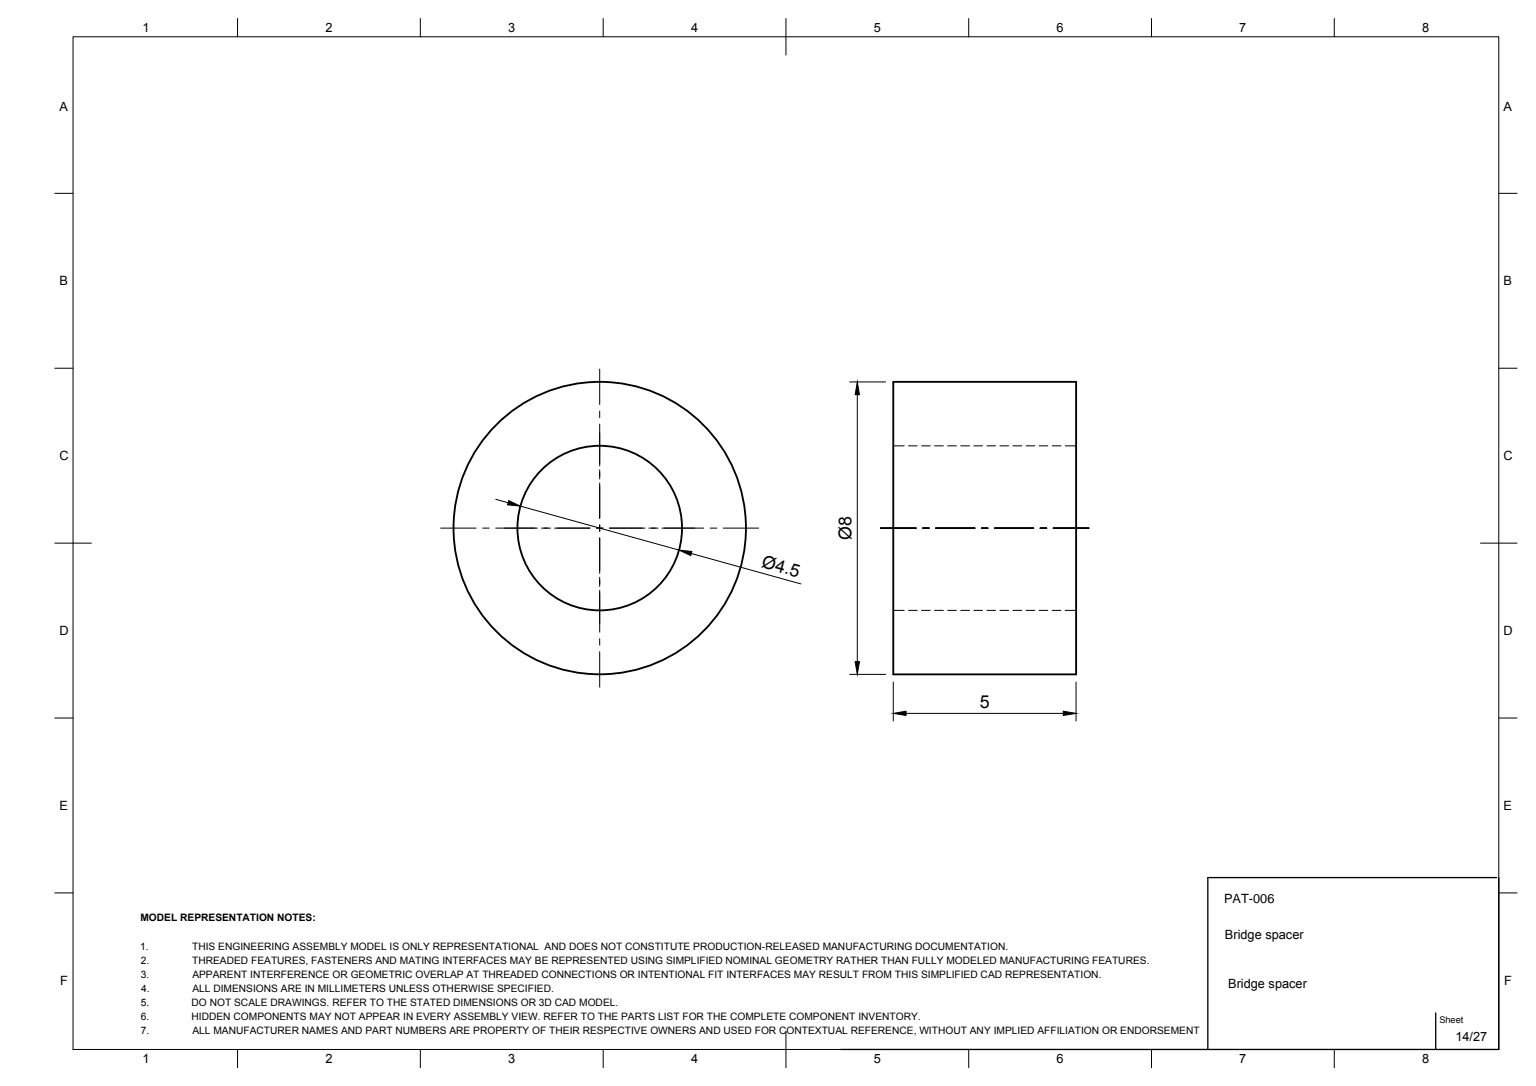
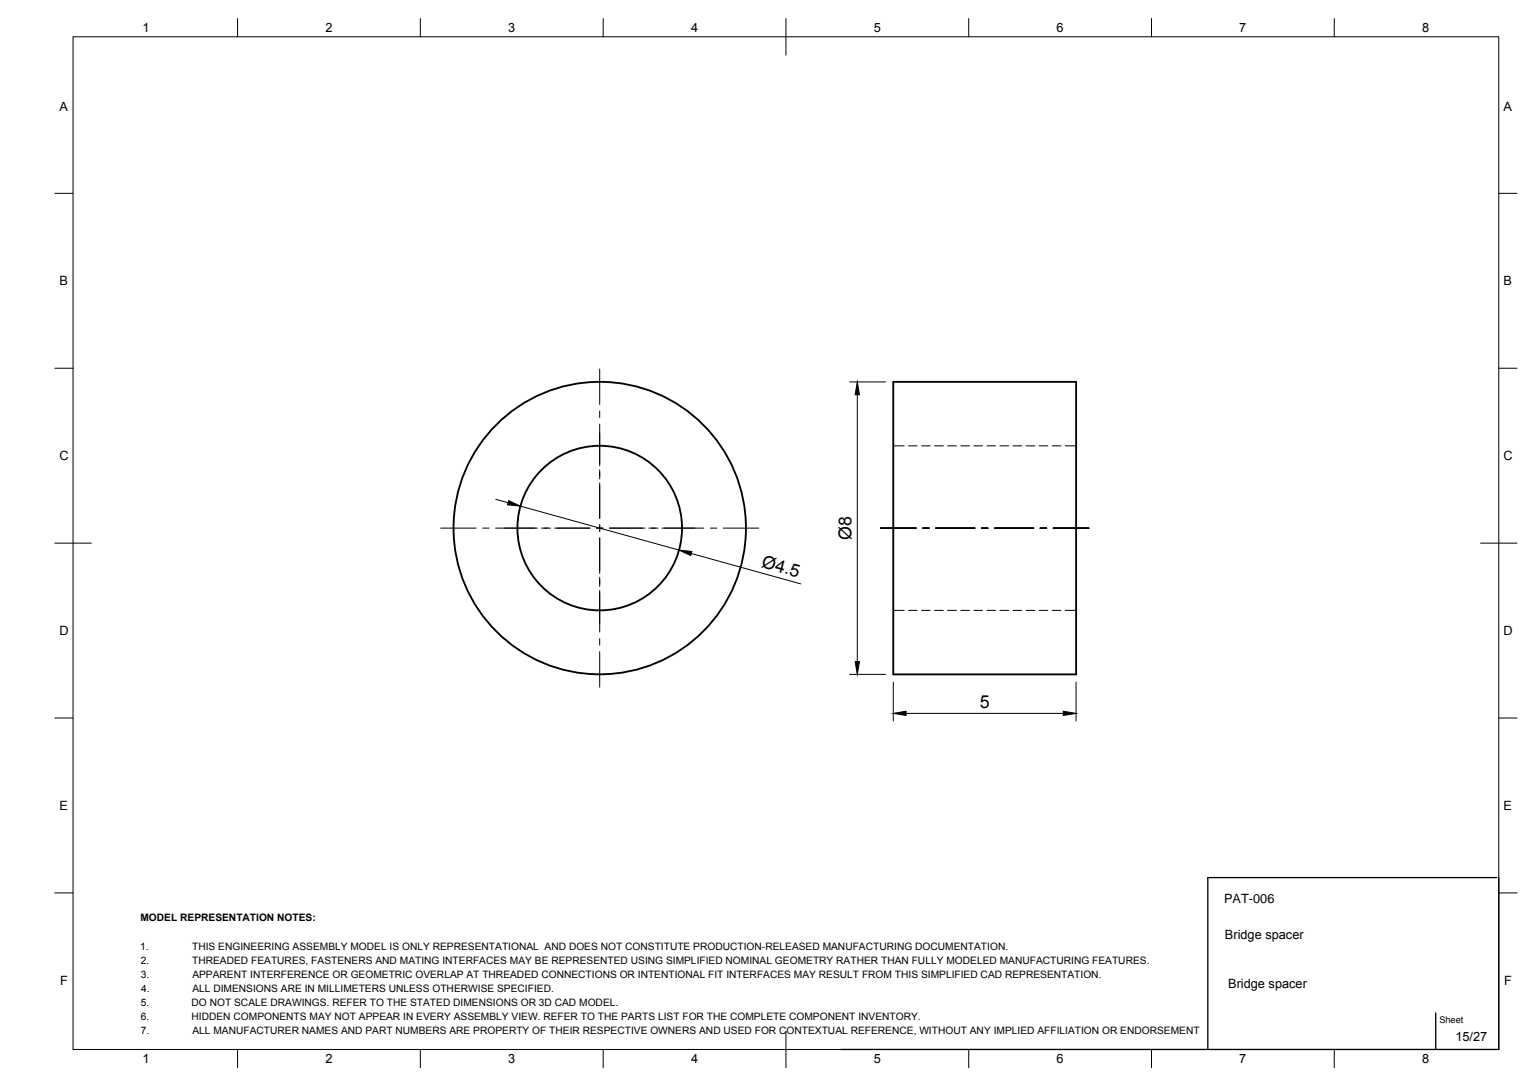
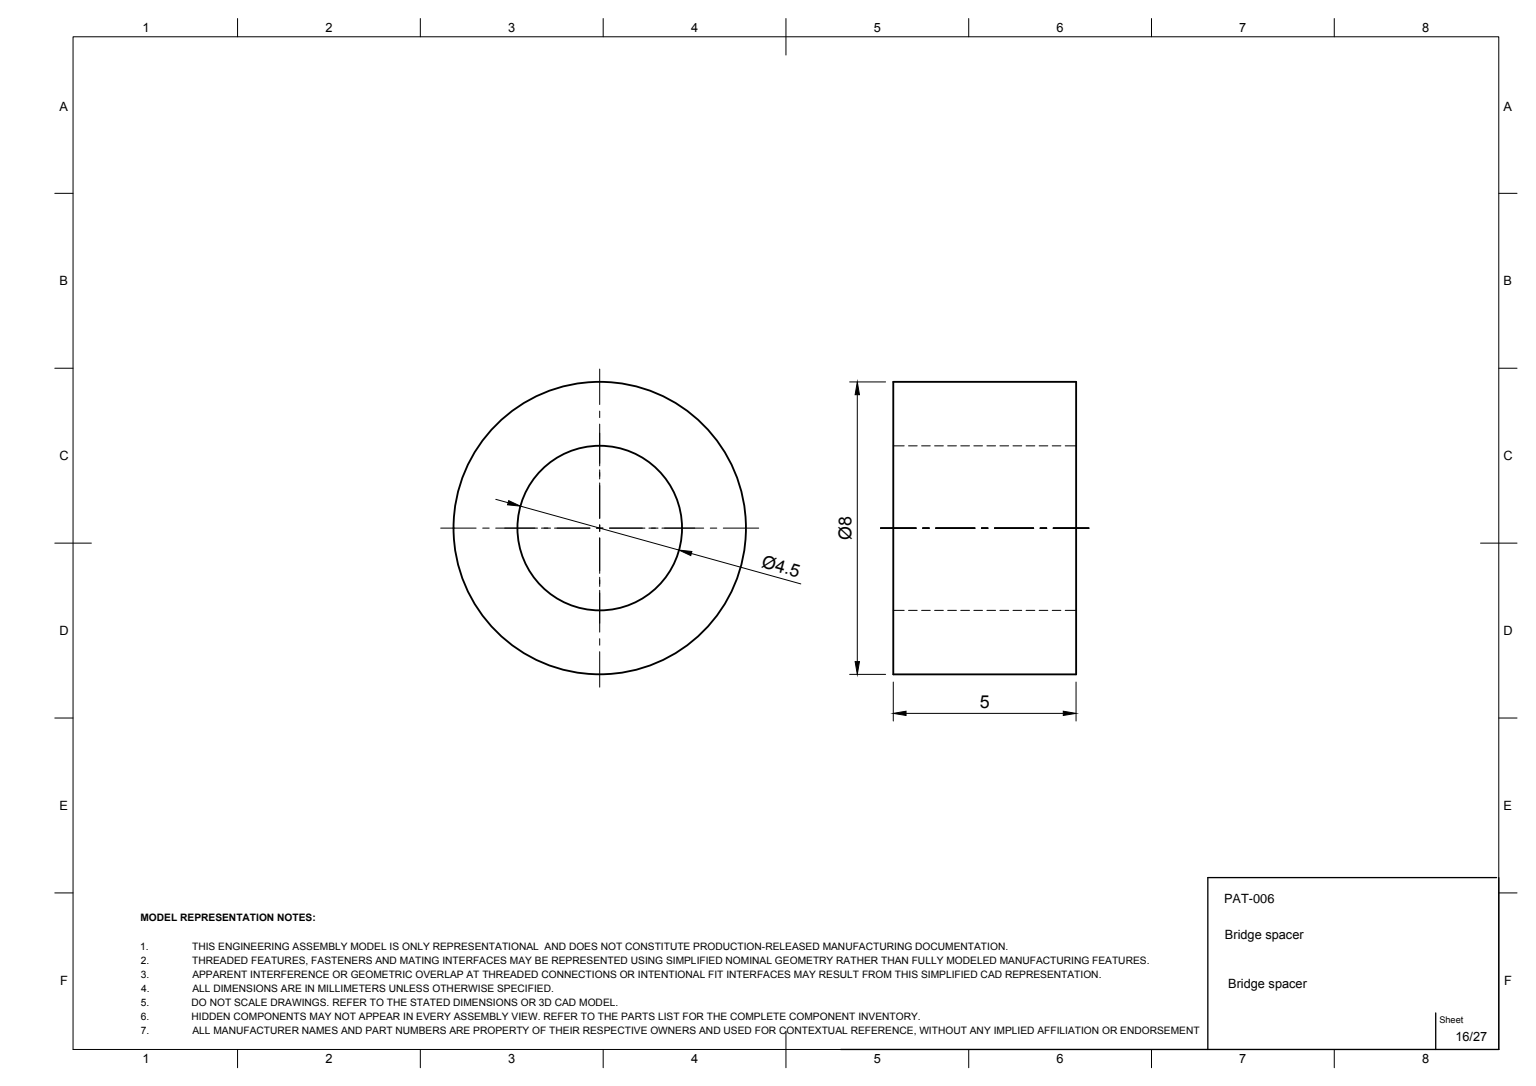
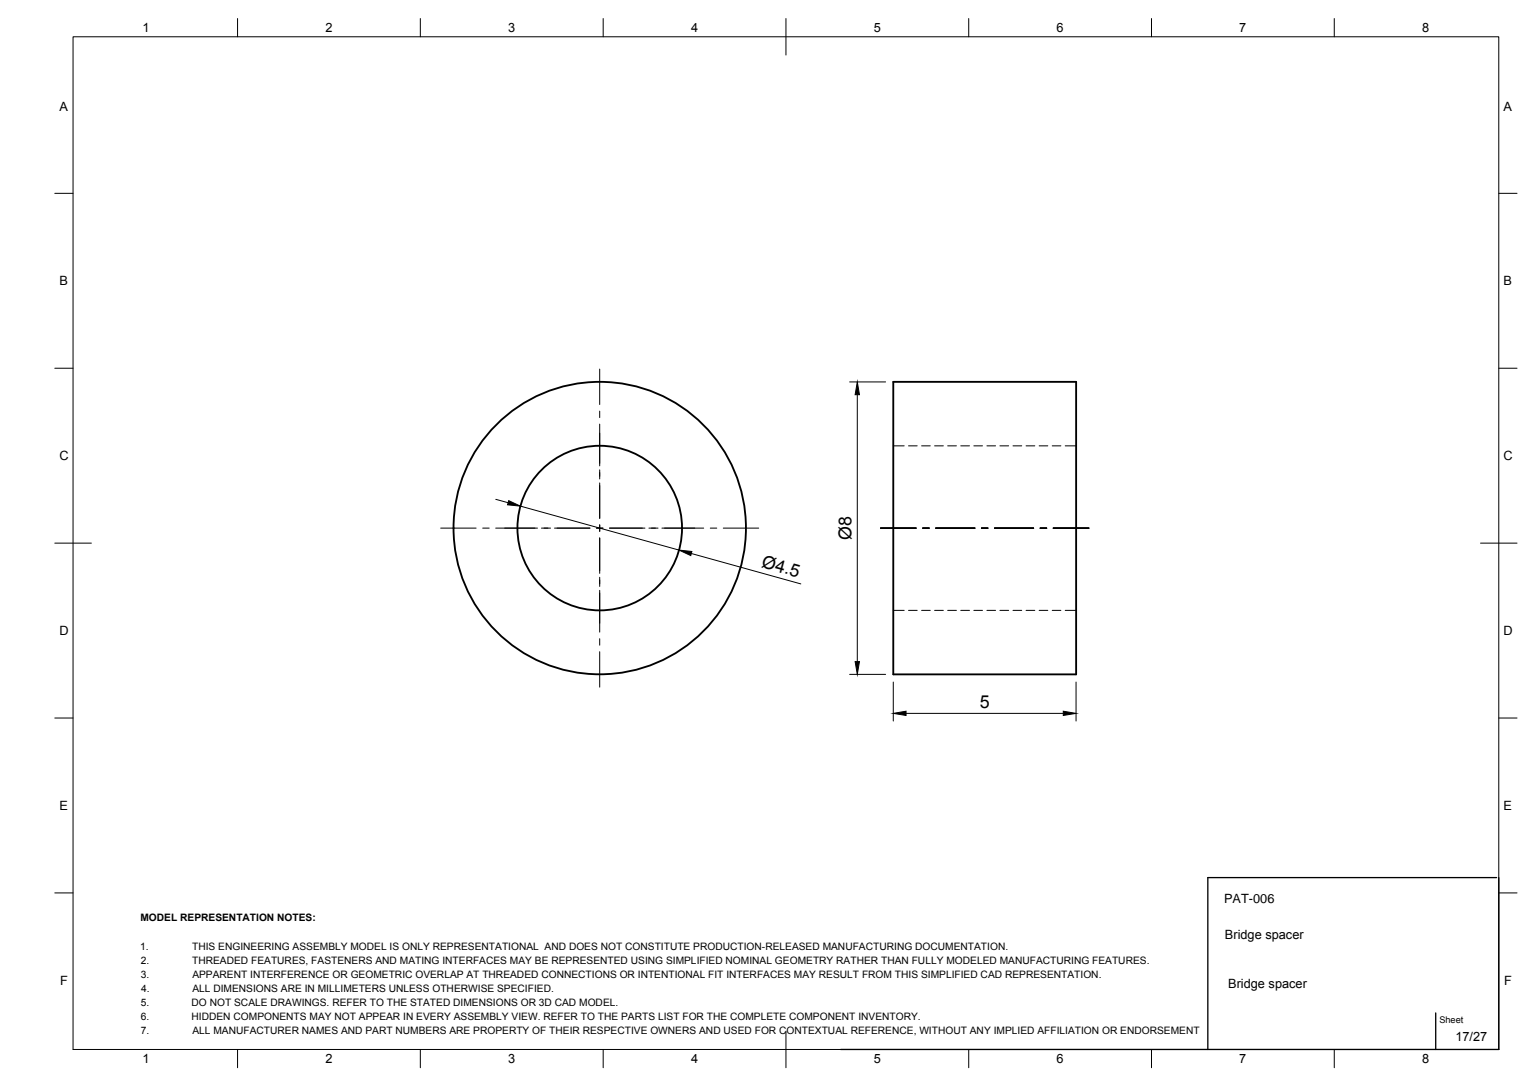
ISO-10303-21;
HEADER;
/* Generated by software containing ST-Developer
 * from STEP Tools, Inc. (www.steptools.com) 
 */

FILE_DESCRIPTION(
/* description */ ('Ball-type isolation valve (generic)'),
/* implementation_level */ '2;1');

FILE_NAME(
/* name */ 'Bridge spacer.step',
/* time_stamp */ '2026-10-27T10:53:05-07:00',
/* author */ (''),
/* organization */ (''),
/* preprocessor_version */ 'ST-DEVELOPER v20.2',
/* originating_system */ 'Autodesk Translation Framework v15.17.0.0',
/* authorisation */ '');

FILE_SCHEMA (('AUTOMOTIVE_DESIGN { 1 0 10303 214 3 1 1 }'));
ENDSEC;

DATA;
#10=MECHANICAL_DESIGN_GEOMETRIC_PRESENTATION_REPRESENTATION('',(#286),#7425);
#234=SHAPE_REPRESENTATION_RELATIONSHIP('SRR','None',#7544,#260);
#260=ADVANCED_BREP_SHAPE_REPRESENTATION('',(#312),#7407);
#286=STYLED_ITEM('',(#7737),#312);
#312=MANIFOLD_SOLID_BREP('Body1',#4091);
#391=FACE_BOUND('',#987,.T.);
#392=FACE_BOUND('',#989,.T.);
#470=PLANE('',#4602);
#471=PLANE('',#4603);
#675=FACE_OUTER_BOUND('',#984,.T.);
#676=FACE_OUTER_BOUND('',#985,.T.);
#677=FACE_OUTER_BOUND('',#986,.T.);
#678=FACE_OUTER_BOUND('',#988,.T.);
#984=EDGE_LOOP('',(#3177,#3178,#3179,#3180));
#985=EDGE_LOOP('',(#3181,#3182,#3183,#3184));
#986=EDGE_LOOP('',(#3185));
#987=EDGE_LOOP('',(#3186));
#988=EDGE_LOOP('',(#3187));
#989=EDGE_LOOP('',(#3188));
#1276=LINE('',#6648,#1584);
#1277=LINE('',#6654,#1585);
#1584=VECTOR('',#5407,0.225);
#1585=VECTOR('',#5414,0.4);
#1871=CIRCLE('',#4597,0.225);
#1872=CIRCLE('',#4598,0.225);
#1873=CIRCLE('',#4600,0.4);
#1874=CIRCLE('',#4601,0.4);
#2091=VERTEX_POINT('',#6645);
#2092=VERTEX_POINT('',#6647);
#2093=VERTEX_POINT('',#6651);
#2094=VERTEX_POINT('',#6653);
#2481=EDGE_CURVE('',#2091,#2091,#1871,.T.);
#2482=EDGE_CURVE('',#2091,#2092,#1276,.T.);
#2483=EDGE_CURVE('',#2092,#2092,#1872,.T.);
#2484=EDGE_CURVE('',#2093,#2093,#1873,.T.);
#2485=EDGE_CURVE('',#2093,#2094,#1277,.T.);
#2486=EDGE_CURVE('',#2094,#2094,#1874,.T.);
#3177=ORIENTED_EDGE('',*,*,#2481,.F.);
#3178=ORIENTED_EDGE('',*,*,#2482,.T.);
#3179=ORIENTED_EDGE('',*,*,#2483,.T.);
#3180=ORIENTED_EDGE('',*,*,#2482,.F.);
#3181=ORIENTED_EDGE('',*,*,#2484,.F.);
#3182=ORIENTED_EDGE('',*,*,#2485,.T.);
#3183=ORIENTED_EDGE('',*,*,#2486,.T.);
#3184=ORIENTED_EDGE('',*,*,#2485,.F.);
#3185=ORIENTED_EDGE('',*,*,#2484,.T.);
#3186=ORIENTED_EDGE('',*,*,#2481,.T.);
#3187=ORIENTED_EDGE('',*,*,#2486,.F.);
#3188=ORIENTED_EDGE('',*,*,#2483,.F.);
#3805=CYLINDRICAL_SURFACE('',#4596,0.225);
#3806=CYLINDRICAL_SURFACE('',#4599,0.4);
#3929=ADVANCED_FACE('',(#675),#3805,.F.);
#3930=ADVANCED_FACE('',(#676),#3806,.T.);
#3931=ADVANCED_FACE('',(#677,#391),#470,.T.);
#3932=ADVANCED_FACE('',(#678,#392),#471,.F.);
#4091=CLOSED_SHELL('',(#3929,#3930,#3931,#3932));
#4595=AXIS2_PLACEMENT_3D('',#6643,#5401,#5402);
#4596=AXIS2_PLACEMENT_3D('',#6644,#5403,#5404);
#4597=AXIS2_PLACEMENT_3D('',#6646,#5405,#5406);
#4598=AXIS2_PLACEMENT_3D('',#6649,#5408,#5409);
#4599=AXIS2_PLACEMENT_3D('',#6650,#5410,#5411);
#4600=AXIS2_PLACEMENT_3D('',#6652,#5412,#5413);
#4601=AXIS2_PLACEMENT_3D('',#6655,#5415,#5416);
#4602=AXIS2_PLACEMENT_3D('',#6656,#5417,#5418);
#4603=AXIS2_PLACEMENT_3D('',#6657,#5419,#5420);
#5401=DIRECTION('axis',(0.,0.,1.));
#5402=DIRECTION('refdir',(1.,0.,0.));
#5403=DIRECTION('center_axis',(0.,0.,1.));
#5404=DIRECTION('ref_axis',(1.,0.,0.));
#5405=DIRECTION('center_axis',(0.,0.,-1.));
#5406=DIRECTION('ref_axis',(1.,0.,0.));
#5407=DIRECTION('',(0.,0.,-1.));
#5408=DIRECTION('center_axis',(0.,0.,-1.));
#5409=DIRECTION('ref_axis',(1.,0.,0.));
#5410=DIRECTION('center_axis',(0.,0.,1.));
#5411=DIRECTION('ref_axis',(1.,0.,0.));
#5412=DIRECTION('center_axis',(0.,0.,1.));
#5413=DIRECTION('ref_axis',(1.,0.,0.));
#5414=DIRECTION('',(0.,0.,-1.));
#5415=DIRECTION('center_axis',(0.,0.,1.));
#5416=DIRECTION('ref_axis',(1.,0.,0.));
#5417=DIRECTION('center_axis',(0.,0.,1.));
#5418=DIRECTION('ref_axis',(1.,0.,0.));
#5419=DIRECTION('center_axis',(0.,0.,1.));
#5420=DIRECTION('ref_axis',(1.,0.,0.));
#6643=CARTESIAN_POINT('',(0.,0.,0.));
#6644=CARTESIAN_POINT('Origin',(-1.3,-1.,7.5));
#6645=CARTESIAN_POINT('',(-1.525,-1.,8.));
#6646=CARTESIAN_POINT('Origin',(-1.3,-1.,8.));
#6647=CARTESIAN_POINT('',(-1.525,-1.,7.5));
#6648=CARTESIAN_POINT('',(-1.525,-1.,7.5));
#6649=CARTESIAN_POINT('Origin',(-1.3,-1.,7.5));
#6650=CARTESIAN_POINT('Origin',(-1.3,-1.,7.5));
#6651=CARTESIAN_POINT('',(-1.7,-1.,8.));
#6652=CARTESIAN_POINT('Origin',(-1.3,-1.,8.));
#6653=CARTESIAN_POINT('',(-1.7,-1.,7.5));
#6654=CARTESIAN_POINT('',(-1.7,-1.,7.5));
#6655=CARTESIAN_POINT('Origin',(-1.3,-1.,7.5));
#6656=CARTESIAN_POINT('Origin',(-1.3,-1.,8.));
#6657=CARTESIAN_POINT('Origin',(-1.3,-1.,7.5));
#7377=UNCERTAINTY_MEASURE_WITH_UNIT(LENGTH_MEASURE(0.001),#7426,
'DISTANCE_ACCURACY_VALUE',
'Maximum model space distance between geometric entities at asserted c
onnectivities');
#7395=UNCERTAINTY_MEASURE_WITH_UNIT(LENGTH_MEASURE(0.001),#7426,
'DISTANCE_ACCURACY_VALUE',
'Maximum model space distance between geometric entities at asserted c
onnectivities');
#7407=(
GEOMETRIC_REPRESENTATION_CONTEXT(3)
GLOBAL_UNCERTAINTY_ASSIGNED_CONTEXT((#7377))
GLOBAL_UNIT_ASSIGNED_CONTEXT((#7426,#7428,#7429))
REPRESENTATION_CONTEXT('','3D')
);
#7425=(
GEOMETRIC_REPRESENTATION_CONTEXT(3)
GLOBAL_UNCERTAINTY_ASSIGNED_CONTEXT((#7395))
GLOBAL_UNIT_ASSIGNED_CONTEXT((#7426,#7428,#7429))
REPRESENTATION_CONTEXT('','3D')
);
#7426=(
LENGTH_UNIT()
NAMED_UNIT(*)
SI_UNIT(.CENTI.,.METRE.)
);
#7428=(
NAMED_UNIT(*)
PLANE_ANGLE_UNIT()
SI_UNIT($,.RADIAN.)
);
#7429=(
NAMED_UNIT(*)
SI_UNIT($,.STERADIAN.)
SOLID_ANGLE_UNIT()
);
#7441=SHAPE_DEFINITION_REPRESENTATION(#7470,#7544);
#7470=PRODUCT_DEFINITION_SHAPE('',$,#7574);
#7544=SHAPE_REPRESENTATION('',(#4595),#7407);
#7562=PRODUCT_DEFINITION_CONTEXT('part definition',#7651,'design');
#7574=PRODUCT_DEFINITION('Bridge spacer','Bridge spacer',#7603,#7562);
#7603=PRODUCT_DEFINITION_FORMATION('',$,#7664);
#7651=APPLICATION_CONTEXT(
'Core Data for Automotive Mechanical Design Process');
#7652=PRODUCT_CONTEXT('part definition',#7651,'mechanical');
#7664=PRODUCT('Bridge spacer','Bridge spacer','Bridge spacer',(#7652));
#7731=COLOUR_RGB('Sky Blue',0.24,0.69,0.87);
#7732=FILL_AREA_STYLE_COLOUR('',#7731);
#7733=FILL_AREA_STYLE('',(#7732));
#7734=SURFACE_STYLE_FILL_AREA(#7733);
#7735=SURFACE_SIDE_STYLE('',(#7734));
#7736=SURFACE_STYLE_USAGE(.BOTH.,#7735);
#7737=PRESENTATION_STYLE_ASSIGNMENT((#7736));
ENDSEC;
END-ISO-10303-21;
